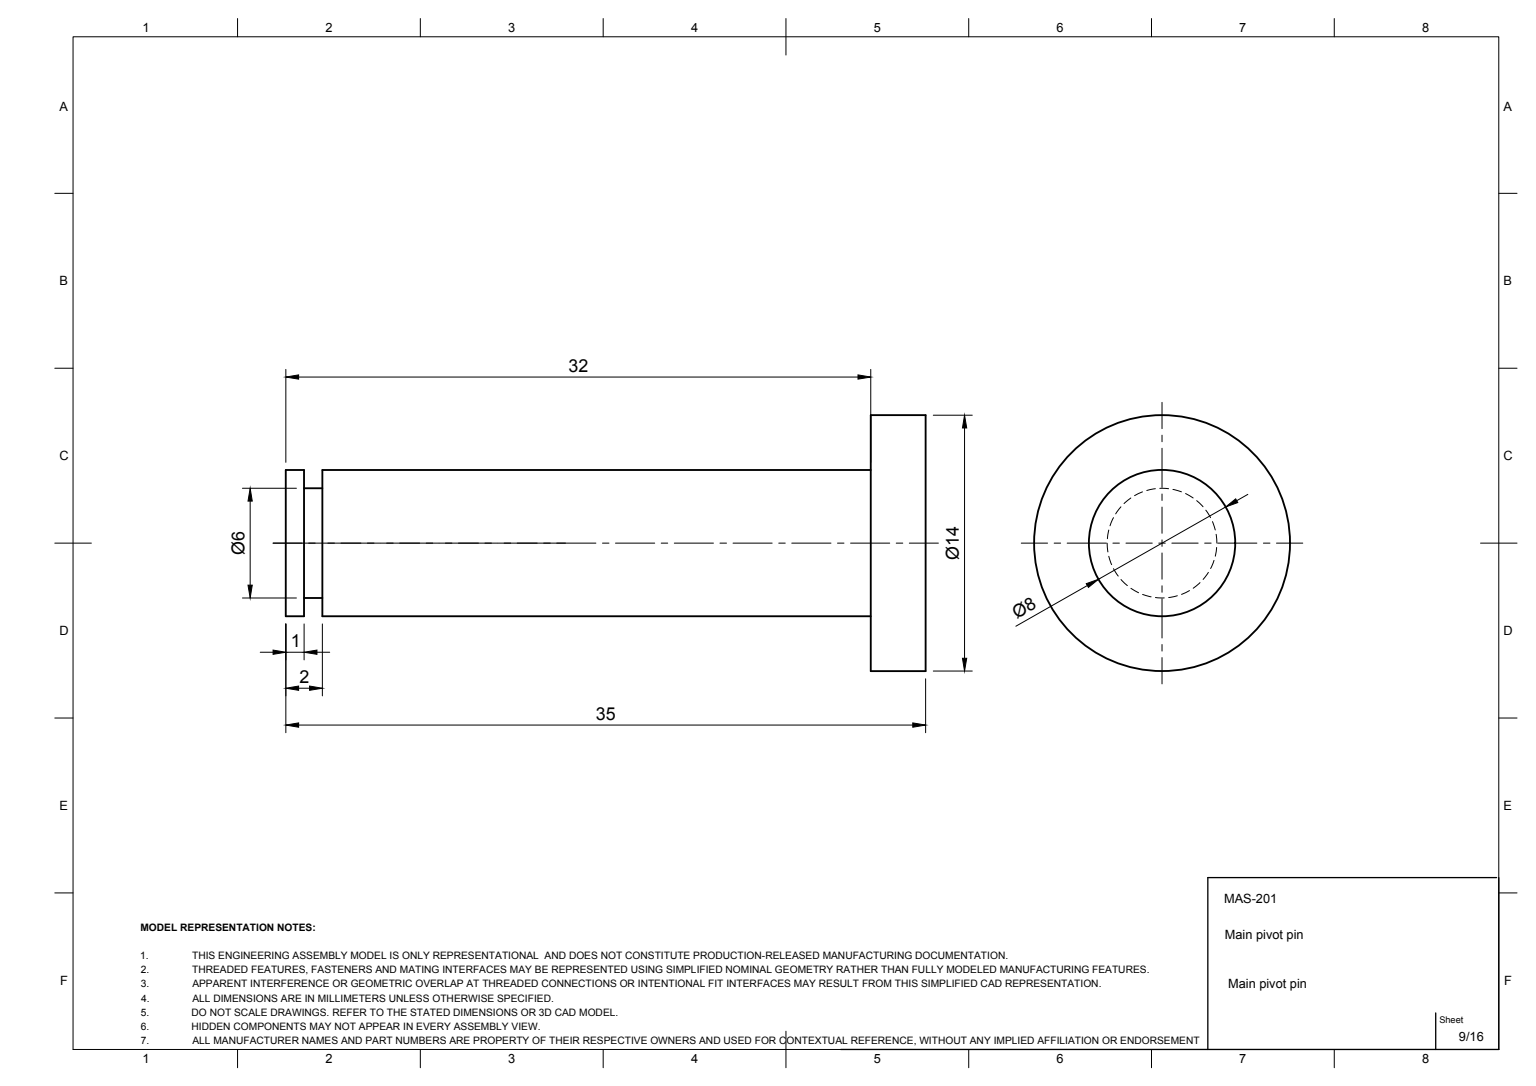
ISO-10303-21;
HEADER;
/* Generated by software containing ST-Developer
 * from STEP Tools, Inc. (www.steptools.com) 
 */

FILE_DESCRIPTION(
/* description */ ('Independent manual two-gate roller-track escapement for nominal30mm d
iameter20mm wide feed rollers. Opposed gates are driven by native capt
ured pin-slot loops with positive curved-slot travel stops at\X\B116de
g. Repeated gate/pin/washer/clip instances, adapted native common bear
ing families, full retaining lips and rotating polymer grip. External 
workpieces, gravity feeder/incline and mount anchors outside assembly.
 No powered-feed compatibility, impact, capacity, safety, force, wear 
or life rating.'),
/* implementation_level */ '2;1');

FILE_NAME(
/* name */ 'Main pivot pin.step',
/* time_stamp */ '2026-11-08T18:43:23-08:00',
/* author */ (''),
/* organization */ (''),
/* preprocessor_version */ 'ST-DEVELOPER v20.2',
/* originating_system */ 'Autodesk Translation Framework v15.17.0.0',
/* authorisation */ '');

FILE_SCHEMA (('AUTOMOTIVE_DESIGN { 1 0 10303 214 3 1 1 }'));
ENDSEC;

DATA;
#10=MECHANICAL_DESIGN_GEOMETRIC_PRESENTATION_REPRESENTATION('',(#460),#19863);
#422=SHAPE_REPRESENTATION_RELATIONSHIP('SRR','None',#19940,#441);
#441=ADVANCED_BREP_SHAPE_REPRESENTATION('',(#479),#19849);
#460=STYLED_ITEM('',(#20042),#479);
#479=MANIFOLD_SOLID_BREP('Body1',#6429);
#830=LINE('',#15803,#1295);
#831=LINE('',#15814,#1296);
#832=LINE('',#15822,#1297);
#833=LINE('',#15826,#1298);
#1295=VECTOR('',#8116,3.);
#1296=VECTOR('',#8131,4.);
#1297=VECTOR('',#8140,7.);
#1298=VECTOR('',#8147,4.);
#1540=CYLINDRICAL_SURFACE('',#6945,3.);
#1541=CYLINDRICAL_SURFACE('',#6952,4.);
#1542=CYLINDRICAL_SURFACE('',#6957,7.);
#1543=CYLINDRICAL_SURFACE('',#6960,4.);
#1662=FACE_BOUND('',#2312,.T.);
#1663=FACE_BOUND('',#2314,.T.);
#1664=FACE_BOUND('',#2317,.T.);
#1906=FACE_OUTER_BOUND('',#2310,.T.);
#1907=FACE_OUTER_BOUND('',#2311,.T.);
#1908=FACE_OUTER_BOUND('',#2313,.T.);
#1909=FACE_OUTER_BOUND('',#2315,.T.);
#1910=FACE_OUTER_BOUND('',#2316,.T.);
#1911=FACE_OUTER_BOUND('',#2318,.T.);
#1912=FACE_OUTER_BOUND('',#2319,.T.);
#1913=FACE_OUTER_BOUND('',#2320,.T.);
#1914=FACE_OUTER_BOUND('',#2321,.T.);
#2310=EDGE_LOOP('',(#5313,#5314,#5315,#5316));
#2311=EDGE_LOOP('',(#5317));
#2312=EDGE_LOOP('',(#5318));
#2313=EDGE_LOOP('',(#5319));
#2314=EDGE_LOOP('',(#5320));
#2315=EDGE_LOOP('',(#5321,#5322,#5323,#5324));
#2316=EDGE_LOOP('',(#5325));
#2317=EDGE_LOOP('',(#5326));
#2318=EDGE_LOOP('',(#5327,#5328,#5329,#5330));
#2319=EDGE_LOOP('',(#5331));
#2320=EDGE_LOOP('',(#5332,#5333,#5334,#5335));
#2321=EDGE_LOOP('',(#5336));
#2546=CIRCLE('',#6946,3.);
#2547=CIRCLE('',#6947,3.);
#2548=CIRCLE('',#6949,4.);
#2549=CIRCLE('',#6951,4.);
#2550=CIRCLE('',#6953,4.);
#2551=CIRCLE('',#6955,7.);
#2552=CIRCLE('',#6956,4.);
#2553=CIRCLE('',#6958,7.);
#3016=VERTEX_POINT('',#15800);
#3017=VERTEX_POINT('',#15802);
#3018=VERTEX_POINT('',#15806);
#3019=VERTEX_POINT('',#15809);
#3020=VERTEX_POINT('',#15812);
#3021=VERTEX_POINT('',#15816);
#3022=VERTEX_POINT('',#15818);
#3023=VERTEX_POINT('',#15821);
#3815=EDGE_CURVE('',#3016,#3016,#2546,.T.);
#3816=EDGE_CURVE('',#3016,#3017,#830,.T.);
#3817=EDGE_CURVE('',#3017,#3017,#2547,.T.);
#3818=EDGE_CURVE('',#3018,#3018,#2548,.T.);
#3819=EDGE_CURVE('',#3019,#3019,#2549,.T.);
#3820=EDGE_CURVE('',#3020,#3020,#2550,.T.);
#3821=EDGE_CURVE('',#3020,#3019,#831,.T.);
#3822=EDGE_CURVE('',#3021,#3021,#2551,.T.);
#3823=EDGE_CURVE('',#3022,#3022,#2552,.T.);
#3824=EDGE_CURVE('',#3021,#3023,#832,.T.);
#3825=EDGE_CURVE('',#3023,#3023,#2553,.T.);
#3826=EDGE_CURVE('',#3018,#3022,#833,.T.);
#5313=ORIENTED_EDGE('',*,*,#3815,.T.);
#5314=ORIENTED_EDGE('',*,*,#3816,.T.);
#5315=ORIENTED_EDGE('',*,*,#3817,.F.);
#5316=ORIENTED_EDGE('',*,*,#3816,.F.);
#5317=ORIENTED_EDGE('',*,*,#3818,.F.);
#5318=ORIENTED_EDGE('',*,*,#3815,.F.);
#5319=ORIENTED_EDGE('',*,*,#3819,.F.);
#5320=ORIENTED_EDGE('',*,*,#3817,.T.);
#5321=ORIENTED_EDGE('',*,*,#3820,.F.);
#5322=ORIENTED_EDGE('',*,*,#3821,.T.);
#5323=ORIENTED_EDGE('',*,*,#3819,.T.);
#5324=ORIENTED_EDGE('',*,*,#3821,.F.);
#5325=ORIENTED_EDGE('',*,*,#3822,.T.);
#5326=ORIENTED_EDGE('',*,*,#3823,.F.);
#5327=ORIENTED_EDGE('',*,*,#3822,.F.);
#5328=ORIENTED_EDGE('',*,*,#3824,.T.);
#5329=ORIENTED_EDGE('',*,*,#3825,.T.);
#5330=ORIENTED_EDGE('',*,*,#3824,.F.);
#5331=ORIENTED_EDGE('',*,*,#3825,.F.);
#5332=ORIENTED_EDGE('',*,*,#3818,.T.);
#5333=ORIENTED_EDGE('',*,*,#3826,.T.);
#5334=ORIENTED_EDGE('',*,*,#3823,.T.);
#5335=ORIENTED_EDGE('',*,*,#3826,.F.);
#5336=ORIENTED_EDGE('',*,*,#3820,.T.);
#6009=PLANE('',#6948);
#6010=PLANE('',#6950);
#6011=PLANE('',#6954);
#6012=PLANE('',#6959);
#6013=PLANE('',#6961);
#6285=ADVANCED_FACE('',(#1906),#1540,.T.);
#6286=ADVANCED_FACE('',(#1907,#1662),#6009,.F.);
#6287=ADVANCED_FACE('',(#1908,#1663),#6010,.F.);
#6288=ADVANCED_FACE('',(#1909),#1541,.T.);
#6289=ADVANCED_FACE('',(#1910,#1664),#6011,.T.);
#6290=ADVANCED_FACE('',(#1911),#1542,.T.);
#6291=ADVANCED_FACE('',(#1912),#6012,.F.);
#6292=ADVANCED_FACE('',(#1913),#1543,.T.);
#6293=ADVANCED_FACE('',(#1914),#6013,.T.);
#6429=CLOSED_SHELL('',(#6285,#6286,#6287,#6288,#6289,#6290,#6291,#6292,
#6293));
#6944=AXIS2_PLACEMENT_3D('',#15798,#8110,#8111);
#6945=AXIS2_PLACEMENT_3D('',#15799,#8112,#8113);
#6946=AXIS2_PLACEMENT_3D('',#15801,#8114,#8115);
#6947=AXIS2_PLACEMENT_3D('',#15804,#8117,#8118);
#6948=AXIS2_PLACEMENT_3D('',#15805,#8119,#8120);
#6949=AXIS2_PLACEMENT_3D('',#15807,#8121,#8122);
#6950=AXIS2_PLACEMENT_3D('',#15808,#8123,#8124);
#6951=AXIS2_PLACEMENT_3D('',#15810,#8125,#8126);
#6952=AXIS2_PLACEMENT_3D('',#15811,#8127,#8128);
#6953=AXIS2_PLACEMENT_3D('',#15813,#8129,#8130);
#6954=AXIS2_PLACEMENT_3D('',#15815,#8132,#8133);
#6955=AXIS2_PLACEMENT_3D('',#15817,#8134,#8135);
#6956=AXIS2_PLACEMENT_3D('',#15819,#8136,#8137);
#6957=AXIS2_PLACEMENT_3D('',#15820,#8138,#8139);
#6958=AXIS2_PLACEMENT_3D('',#15823,#8141,#8142);
#6959=AXIS2_PLACEMENT_3D('',#15824,#8143,#8144);
#6960=AXIS2_PLACEMENT_3D('',#15825,#8145,#8146);
#6961=AXIS2_PLACEMENT_3D('',#15827,#8148,#8149);
#8110=DIRECTION('axis',(0.,0.,1.));
#8111=DIRECTION('refdir',(1.,0.,0.));
#8112=DIRECTION('center_axis',(0.,0.,1.));
#8113=DIRECTION('ref_axis',(1.,0.,0.));
#8114=DIRECTION('center_axis',(0.,0.,1.));
#8115=DIRECTION('ref_axis',(1.,0.,0.));
#8116=DIRECTION('',(0.,0.,1.));
#8117=DIRECTION('center_axis',(0.,0.,1.));
#8118=DIRECTION('ref_axis',(1.,0.,0.));
#8119=DIRECTION('center_axis',(0.,0.,-1.));
#8120=DIRECTION('ref_axis',(-1.,0.,0.));
#8121=DIRECTION('center_axis',(0.,0.,-1.));
#8122=DIRECTION('ref_axis',(1.,0.,0.));
#8123=DIRECTION('center_axis',(0.,0.,1.));
#8124=DIRECTION('ref_axis',(1.,0.,0.));
#8125=DIRECTION('center_axis',(0.,0.,1.));
#8126=DIRECTION('ref_axis',(1.,0.,0.));
#8127=DIRECTION('center_axis',(0.,0.,1.));
#8128=DIRECTION('ref_axis',(1.,0.,0.));
#8129=DIRECTION('center_axis',(0.,0.,1.));
#8130=DIRECTION('ref_axis',(1.,0.,0.));
#8131=DIRECTION('',(0.,0.,-1.));
#8132=DIRECTION('center_axis',(0.,0.,1.));
#8133=DIRECTION('ref_axis',(1.,0.,0.));
#8134=DIRECTION('center_axis',(0.,0.,1.));
#8135=DIRECTION('ref_axis',(1.,0.,0.));
#8136=DIRECTION('center_axis',(0.,0.,1.));
#8137=DIRECTION('ref_axis',(1.,0.,0.));
#8138=DIRECTION('center_axis',(0.,0.,1.));
#8139=DIRECTION('ref_axis',(1.,0.,0.));
#8140=DIRECTION('',(0.,0.,-1.));
#8141=DIRECTION('center_axis',(0.,0.,1.));
#8142=DIRECTION('ref_axis',(1.,0.,0.));
#8143=DIRECTION('center_axis',(0.,0.,1.));
#8144=DIRECTION('ref_axis',(1.,0.,0.));
#8145=DIRECTION('center_axis',(0.,0.,1.));
#8146=DIRECTION('ref_axis',(1.,0.,0.));
#8147=DIRECTION('',(0.,0.,-1.));
#8148=DIRECTION('center_axis',(0.,0.,1.));
#8149=DIRECTION('ref_axis',(1.,0.,0.));
#15798=CARTESIAN_POINT('',(0.,0.,0.));
#15799=CARTESIAN_POINT('Origin',(0.,0.,30.5));
#15800=CARTESIAN_POINT('',(-3.,-3.67394039744206E-16,30.));
#15801=CARTESIAN_POINT('Origin',(0.,0.,30.));
#15802=CARTESIAN_POINT('',(-3.,-3.67394039744206E-16,31.));
#15803=CARTESIAN_POINT('',(-3.,-3.67394039744206E-16,30.5));
#15804=CARTESIAN_POINT('Origin',(0.,0.,31.));
#15805=CARTESIAN_POINT('Origin',(7.,0.,30.));
#15806=CARTESIAN_POINT('',(-4.,4.89858719658941E-16,30.));
#15807=CARTESIAN_POINT('Origin',(0.,0.,30.));
#15808=CARTESIAN_POINT('Origin',(3.,0.,31.));
#15809=CARTESIAN_POINT('',(-4.,-4.89858719658941E-16,31.));
#15810=CARTESIAN_POINT('Origin',(0.,0.,31.));
#15811=CARTESIAN_POINT('Origin',(0.,0.,0.));
#15812=CARTESIAN_POINT('',(-4.,-4.89858719658941E-16,32.));
#15813=CARTESIAN_POINT('Origin',(0.,0.,32.));
#15814=CARTESIAN_POINT('',(-4.,-4.89858719658941E-16,0.));
#15815=CARTESIAN_POINT('Origin',(0.,0.,0.));
#15816=CARTESIAN_POINT('',(-7.,-8.57252759403147E-16,0.));
#15817=CARTESIAN_POINT('Origin',(0.,0.,0.));
#15818=CARTESIAN_POINT('',(-4.,-4.89858719658941E-16,0.));
#15819=CARTESIAN_POINT('Origin',(0.,0.,0.));
#15820=CARTESIAN_POINT('Origin',(0.,0.,-3.));
#15821=CARTESIAN_POINT('',(-7.,-8.57252759403147E-16,-3.));
#15822=CARTESIAN_POINT('',(-7.,-8.57252759403147E-16,-3.));
#15823=CARTESIAN_POINT('Origin',(0.,0.,-3.));
#15824=CARTESIAN_POINT('Origin',(0.,0.,-3.));
#15825=CARTESIAN_POINT('Origin',(0.,0.,0.));
#15826=CARTESIAN_POINT('',(-4.,-4.89858719658941E-16,0.));
#15827=CARTESIAN_POINT('Origin',(0.,0.,32.));
#19828=UNCERTAINTY_MEASURE_WITH_UNIT(LENGTH_MEASURE(0.01),#19864,
'DISTANCE_ACCURACY_VALUE',
'Maximum model space distance between geometric entities at asserted c
onnectivities');
#19842=UNCERTAINTY_MEASURE_WITH_UNIT(LENGTH_MEASURE(0.01),#19864,
'DISTANCE_ACCURACY_VALUE',
'Maximum model space distance between geometric entities at asserted c
onnectivities');
#19849=(
GEOMETRIC_REPRESENTATION_CONTEXT(3)
GLOBAL_UNCERTAINTY_ASSIGNED_CONTEXT((#19828))
GLOBAL_UNIT_ASSIGNED_CONTEXT((#19864,#19866,#19867))
REPRESENTATION_CONTEXT('','3D')
);
#19863=(
GEOMETRIC_REPRESENTATION_CONTEXT(3)
GLOBAL_UNCERTAINTY_ASSIGNED_CONTEXT((#19842))
GLOBAL_UNIT_ASSIGNED_CONTEXT((#19864,#19866,#19867))
REPRESENTATION_CONTEXT('','3D')
);
#19864=(
LENGTH_UNIT()
NAMED_UNIT(*)
SI_UNIT(.MILLI.,.METRE.)
);
#19866=(
NAMED_UNIT(*)
PLANE_ANGLE_UNIT()
SI_UNIT($,.RADIAN.)
);
#19867=(
NAMED_UNIT(*)
SI_UNIT($,.STERADIAN.)
SOLID_ANGLE_UNIT()
);
#19874=SHAPE_DEFINITION_REPRESENTATION(#19894,#19940);
#19894=PRODUCT_DEFINITION_SHAPE('',$,#19961);
#19940=SHAPE_REPRESENTATION('',(#6944),#19849);
#19954=PRODUCT_DEFINITION_CONTEXT('part definition',#20016,'design');
#19961=PRODUCT_DEFINITION('Main pivot pin','Main pivot pin',#19981,#19954);
#19981=PRODUCT_DEFINITION_FORMATION('',$,#20024);
#20016=APPLICATION_CONTEXT(
'Core Data for Automotive Mechanical Design Process');
#20017=PRODUCT_CONTEXT('part definition',#20016,'mechanical');
#20024=PRODUCT('Main pivot pin','Main pivot pin',$,(#20017));
#20042=PRESENTATION_STYLE_ASSIGNMENT((#20049));
#20049=SURFACE_STYLE_USAGE(.BOTH.,#20056);
#20056=SURFACE_SIDE_STYLE('',(#20063));
#20063=SURFACE_STYLE_FILL_AREA(#20070);
#20070=FILL_AREA_STYLE('Gray',(#20077));
#20077=FILL_AREA_STYLE_COLOUR('Gray',#20084);
#20084=COLOUR_RGB('Gray',0.407843137254902,0.447058823529412,0.498039215686275);
ENDSEC;
END-ISO-10303-21;
